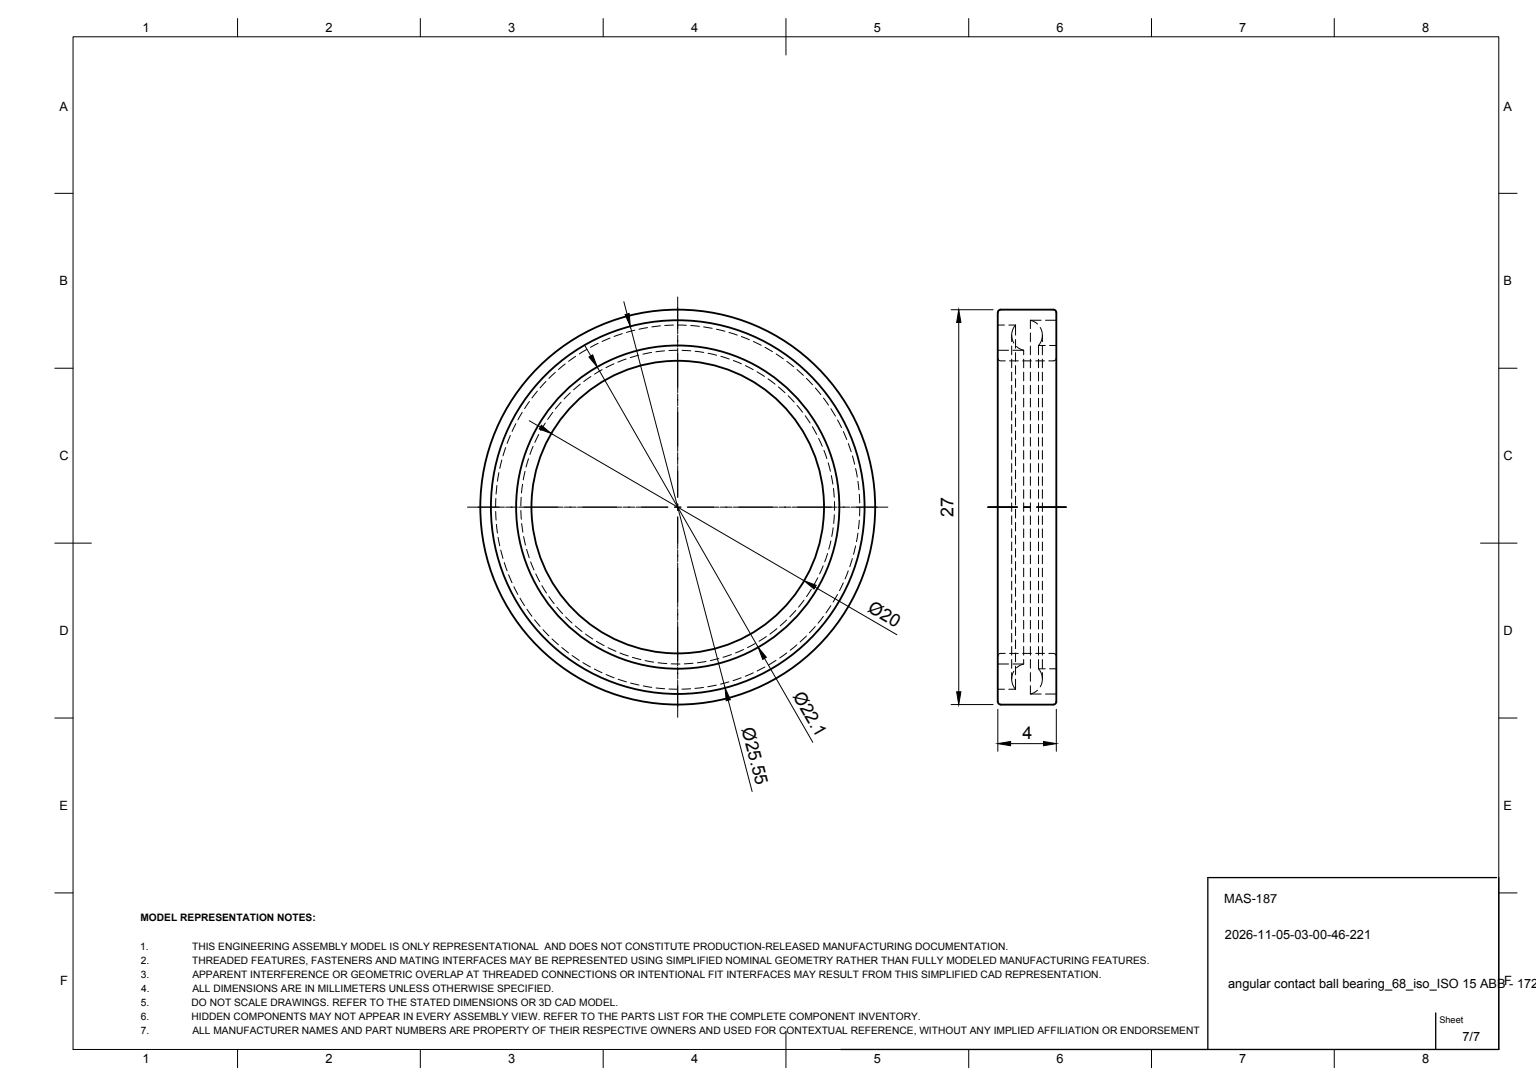
ISO-10303-21;
HEADER;
/* Generated by software containing ST-Developer
 * from STEP Tools, Inc. (www.steptools.com) 
 */

FILE_DESCRIPTION(
/* description */ ('STEP AP214'),
/* implementation_level */ '2;1');

FILE_NAME(
/* name */ 'angular contact ball bearing_68_iso_ISO 15 ABB - 1720 - 28,SI,NC,28_6_8.step',
/* time_stamp */ '2026-11-04T19:00:26-08:00',
/* author */ (''),
/* organization */ (''),
/* preprocessor_version */ 'ST-DEVELOPER v20.2',
/* originating_system */ 'Autodesk Translation Framework v15.17.0.0',
/* authorisation */ '');

FILE_SCHEMA (('AUTOMOTIVE_DESIGN { 1 0 10303 214 3 1 1 }'));
ENDSEC;

DATA;
#10=MECHANICAL_DESIGN_GEOMETRIC_PRESENTATION_REPRESENTATION('',(#274),#5689);
#248=TOROIDAL_SURFACE('',#3187,13.3,0.200000000000003);
#249=TOROIDAL_SURFACE('',#3193,13.3,0.200000000000003);
#250=TOROIDAL_SURFACE('',#3204,11.75,1.05);
#251=TOROIDAL_SURFACE('',#3208,10.2,0.200000000000003);
#252=TOROIDAL_SURFACE('',#3214,10.2,0.200000000000003);
#253=TOROIDAL_SURFACE('',#3223,11.75,1.05);
#260=SHAPE_REPRESENTATION_RELATIONSHIP('SRR','None',#5761,#267);
#267=ADVANCED_BREP_SHAPE_REPRESENTATION('',(#281),#5685);
#274=STYLED_ITEM('',(#5805),#281);
#281=MANIFOLD_SOLID_BREP('Body1',#2964);
#331=FACE_BOUND('',#748,.T.);
#332=FACE_BOUND('',#750,.T.);
#333=FACE_BOUND('',#752,.T.);
#334=FACE_BOUND('',#754,.T.);
#411=PLANE('',#3225);
#412=PLANE('',#3226);
#413=PLANE('',#3227);
#414=PLANE('',#3228);
#530=FACE_OUTER_BOUND('',#735,.T.);
#531=FACE_OUTER_BOUND('',#736,.T.);
#532=FACE_OUTER_BOUND('',#737,.T.);
#533=FACE_OUTER_BOUND('',#738,.T.);
#534=FACE_OUTER_BOUND('',#739,.T.);
#535=FACE_OUTER_BOUND('',#740,.T.);
#536=FACE_OUTER_BOUND('',#741,.T.);
#537=FACE_OUTER_BOUND('',#742,.T.);
#538=FACE_OUTER_BOUND('',#743,.T.);
#539=FACE_OUTER_BOUND('',#744,.T.);
#540=FACE_OUTER_BOUND('',#745,.T.);
#541=FACE_OUTER_BOUND('',#746,.T.);
#542=FACE_OUTER_BOUND('',#747,.T.);
#543=FACE_OUTER_BOUND('',#749,.T.);
#544=FACE_OUTER_BOUND('',#751,.T.);
#545=FACE_OUTER_BOUND('',#753,.T.);
#735=EDGE_LOOP('',(#2472,#2473,#2474,#2475));
#736=EDGE_LOOP('',(#2476,#2477,#2478,#2479));
#737=EDGE_LOOP('',(#2480,#2481,#2482,#2483));
#738=EDGE_LOOP('',(#2484,#2485,#2486,#2487,#2488));
#739=EDGE_LOOP('',(#2489,#2490,#2491,#2492,#2493));
#740=EDGE_LOOP('',(#2494,#2495,#2496,#2497,#2498,#2499));
#741=EDGE_LOOP('',(#2500,#2501,#2502,#2503));
#742=EDGE_LOOP('',(#2504,#2505,#2506,#2507));
#743=EDGE_LOOP('',(#2508,#2509,#2510,#2511));
#744=EDGE_LOOP('',(#2512,#2513,#2514,#2515,#2516));
#745=EDGE_LOOP('',(#2517,#2518,#2519,#2520,#2521));
#746=EDGE_LOOP('',(#2522,#2523,#2524,#2525,#2526,#2527));
#747=EDGE_LOOP('',(#2528));
#748=EDGE_LOOP('',(#2529));
#749=EDGE_LOOP('',(#2530));
#750=EDGE_LOOP('',(#2531));
#751=EDGE_LOOP('',(#2532));
#752=EDGE_LOOP('',(#2533));
#753=EDGE_LOOP('',(#2534));
#754=EDGE_LOOP('',(#2535));
#1000=LINE('',#4725,#1231);
#1001=LINE('',#4735,#1232);
#1002=LINE('',#4745,#1233);
#1003=LINE('',#4761,#1234);
#1004=LINE('',#4769,#1235);
#1005=LINE('',#4775,#1236);
#1231=VECTOR('',#3843,13.5);
#1232=VECTOR('',#3856,12.775);
#1233=VECTOR('',#3867,12.45);
#1234=VECTOR('',#3888,10.);
#1235=VECTOR('',#3899,11.05);
#1236=VECTOR('',#3906,10.725);
#1328=CIRCLE('',#3188,13.3);
#1329=CIRCLE('',#3189,0.200000000000003);
#1330=CIRCLE('',#3190,13.5);
#1331=CIRCLE('',#3192,13.5);
#1332=CIRCLE('',#3194,0.200000000000003);
#1333=CIRCLE('',#3195,13.3);
#1334=CIRCLE('',#3197,12.775);
#1335=CIRCLE('',#3198,12.775);
#1336=CIRCLE('',#3199,12.775);
#1337=CIRCLE('',#3201,12.45);
#1338=CIRCLE('',#3202,12.45);
#1339=CIRCLE('',#3203,12.45);
#1340=CIRCLE('',#3205,11.05);
#1341=CIRCLE('',#3206,1.05);
#1342=CIRCLE('',#3207,11.05);
#1343=CIRCLE('',#3209,10.2);
#1344=CIRCLE('',#3210,0.200000000000003);
#1345=CIRCLE('',#3211,10.);
#1346=CIRCLE('',#3213,10.);
#1347=CIRCLE('',#3215,0.200000000000003);
#1348=CIRCLE('',#3216,10.2);
#1349=CIRCLE('',#3218,11.05);
#1350=CIRCLE('',#3220,10.725);
#1351=CIRCLE('',#3221,10.725);
#1352=CIRCLE('',#3222,10.725);
#1353=CIRCLE('',#3224,1.05);
#1543=VERTEX_POINT('',#4718);
#1544=VERTEX_POINT('',#4720);
#1545=VERTEX_POINT('',#4724);
#1546=VERTEX_POINT('',#4728);
#1547=VERTEX_POINT('',#4732);
#1548=VERTEX_POINT('',#4734);
#1549=VERTEX_POINT('',#4736);
#1550=VERTEX_POINT('',#4740);
#1551=VERTEX_POINT('',#4741);
#1552=VERTEX_POINT('',#4744);
#1553=VERTEX_POINT('',#4748);
#1554=VERTEX_POINT('',#4749);
#1555=VERTEX_POINT('',#4754);
#1556=VERTEX_POINT('',#4756);
#1557=VERTEX_POINT('',#4760);
#1558=VERTEX_POINT('',#4764);
#1559=VERTEX_POINT('',#4768);
#1560=VERTEX_POINT('',#4772);
#1561=VERTEX_POINT('',#4774);
#1562=VERTEX_POINT('',#4776);
#1864=EDGE_CURVE('',#1543,#1543,#1328,.T.);
#1865=EDGE_CURVE('',#1543,#1544,#1329,.T.);
#1866=EDGE_CURVE('',#1544,#1544,#1330,.T.);
#1867=EDGE_CURVE('',#1544,#1545,#1000,.T.);
#1868=EDGE_CURVE('',#1545,#1545,#1331,.T.);
#1869=EDGE_CURVE('',#1545,#1546,#1332,.T.);
#1870=EDGE_CURVE('',#1546,#1546,#1333,.T.);
#1871=EDGE_CURVE('',#1547,#1547,#1334,.T.);
#1872=EDGE_CURVE('',#1547,#1548,#1001,.T.);
#1873=EDGE_CURVE('',#1549,#1548,#1335,.T.);
#1874=EDGE_CURVE('',#1548,#1549,#1336,.T.);
#1875=EDGE_CURVE('',#1550,#1551,#1337,.T.);
#1876=EDGE_CURVE('',#1551,#1550,#1338,.T.);
#1877=EDGE_CURVE('',#1551,#1552,#1002,.T.);
#1878=EDGE_CURVE('',#1552,#1552,#1339,.T.);
#1879=EDGE_CURVE('',#1553,#1554,#1340,.T.);
#1880=EDGE_CURVE('',#1554,#1549,#1341,.T.);
#1881=EDGE_CURVE('',#1554,#1553,#1342,.T.);
#1882=EDGE_CURVE('',#1555,#1555,#1343,.T.);
#1883=EDGE_CURVE('',#1555,#1556,#1344,.T.);
#1884=EDGE_CURVE('',#1556,#1556,#1345,.T.);
#1885=EDGE_CURVE('',#1556,#1557,#1003,.T.);
#1886=EDGE_CURVE('',#1557,#1557,#1346,.T.);
#1887=EDGE_CURVE('',#1557,#1558,#1347,.T.);
#1888=EDGE_CURVE('',#1558,#1558,#1348,.T.);
#1889=EDGE_CURVE('',#1553,#1559,#1004,.T.);
#1890=EDGE_CURVE('',#1559,#1559,#1349,.T.);
#1891=EDGE_CURVE('',#1560,#1560,#1350,.T.);
#1892=EDGE_CURVE('',#1560,#1561,#1005,.T.);
#1893=EDGE_CURVE('',#1562,#1561,#1351,.T.);
#1894=EDGE_CURVE('',#1561,#1562,#1352,.T.);
#1895=EDGE_CURVE('',#1550,#1562,#1353,.T.);
#2472=ORIENTED_EDGE('',*,*,#1864,.F.);
#2473=ORIENTED_EDGE('',*,*,#1865,.T.);
#2474=ORIENTED_EDGE('',*,*,#1866,.T.);
#2475=ORIENTED_EDGE('',*,*,#1865,.F.);
#2476=ORIENTED_EDGE('',*,*,#1866,.F.);
#2477=ORIENTED_EDGE('',*,*,#1867,.T.);
#2478=ORIENTED_EDGE('',*,*,#1868,.T.);
#2479=ORIENTED_EDGE('',*,*,#1867,.F.);
#2480=ORIENTED_EDGE('',*,*,#1868,.F.);
#2481=ORIENTED_EDGE('',*,*,#1869,.T.);
#2482=ORIENTED_EDGE('',*,*,#1870,.T.);
#2483=ORIENTED_EDGE('',*,*,#1869,.F.);
#2484=ORIENTED_EDGE('',*,*,#1871,.F.);
#2485=ORIENTED_EDGE('',*,*,#1872,.T.);
#2486=ORIENTED_EDGE('',*,*,#1873,.F.);
#2487=ORIENTED_EDGE('',*,*,#1874,.F.);
#2488=ORIENTED_EDGE('',*,*,#1872,.F.);
#2489=ORIENTED_EDGE('',*,*,#1875,.F.);
#2490=ORIENTED_EDGE('',*,*,#1876,.F.);
#2491=ORIENTED_EDGE('',*,*,#1877,.T.);
#2492=ORIENTED_EDGE('',*,*,#1878,.T.);
#2493=ORIENTED_EDGE('',*,*,#1877,.F.);
#2494=ORIENTED_EDGE('',*,*,#1879,.T.);
#2495=ORIENTED_EDGE('',*,*,#1880,.T.);
#2496=ORIENTED_EDGE('',*,*,#1873,.T.);
#2497=ORIENTED_EDGE('',*,*,#1874,.T.);
#2498=ORIENTED_EDGE('',*,*,#1880,.F.);
#2499=ORIENTED_EDGE('',*,*,#1881,.T.);
#2500=ORIENTED_EDGE('',*,*,#1882,.F.);
#2501=ORIENTED_EDGE('',*,*,#1883,.T.);
#2502=ORIENTED_EDGE('',*,*,#1884,.T.);
#2503=ORIENTED_EDGE('',*,*,#1883,.F.);
#2504=ORIENTED_EDGE('',*,*,#1884,.F.);
#2505=ORIENTED_EDGE('',*,*,#1885,.T.);
#2506=ORIENTED_EDGE('',*,*,#1886,.T.);
#2507=ORIENTED_EDGE('',*,*,#1885,.F.);
#2508=ORIENTED_EDGE('',*,*,#1886,.F.);
#2509=ORIENTED_EDGE('',*,*,#1887,.T.);
#2510=ORIENTED_EDGE('',*,*,#1888,.T.);
#2511=ORIENTED_EDGE('',*,*,#1887,.F.);
#2512=ORIENTED_EDGE('',*,*,#1879,.F.);
#2513=ORIENTED_EDGE('',*,*,#1889,.T.);
#2514=ORIENTED_EDGE('',*,*,#1890,.T.);
#2515=ORIENTED_EDGE('',*,*,#1889,.F.);
#2516=ORIENTED_EDGE('',*,*,#1881,.F.);
#2517=ORIENTED_EDGE('',*,*,#1891,.F.);
#2518=ORIENTED_EDGE('',*,*,#1892,.T.);
#2519=ORIENTED_EDGE('',*,*,#1893,.F.);
#2520=ORIENTED_EDGE('',*,*,#1894,.F.);
#2521=ORIENTED_EDGE('',*,*,#1892,.F.);
#2522=ORIENTED_EDGE('',*,*,#1875,.T.);
#2523=ORIENTED_EDGE('',*,*,#1876,.T.);
#2524=ORIENTED_EDGE('',*,*,#1895,.T.);
#2525=ORIENTED_EDGE('',*,*,#1893,.T.);
#2526=ORIENTED_EDGE('',*,*,#1894,.T.);
#2527=ORIENTED_EDGE('',*,*,#1895,.F.);
#2528=ORIENTED_EDGE('',*,*,#1891,.T.);
#2529=ORIENTED_EDGE('',*,*,#1888,.F.);
#2530=ORIENTED_EDGE('',*,*,#1890,.F.);
#2531=ORIENTED_EDGE('',*,*,#1882,.T.);
#2532=ORIENTED_EDGE('',*,*,#1864,.T.);
#2533=ORIENTED_EDGE('',*,*,#1878,.F.);
#2534=ORIENTED_EDGE('',*,*,#1870,.F.);
#2535=ORIENTED_EDGE('',*,*,#1871,.T.);
#2788=CYLINDRICAL_SURFACE('',#3191,13.5);
#2789=CYLINDRICAL_SURFACE('',#3196,12.775);
#2790=CYLINDRICAL_SURFACE('',#3200,12.45);
#2791=CYLINDRICAL_SURFACE('',#3212,10.);
#2792=CYLINDRICAL_SURFACE('',#3217,11.05);
#2793=CYLINDRICAL_SURFACE('',#3219,10.725);
#2890=ADVANCED_FACE('',(#530),#248,.T.);
#2891=ADVANCED_FACE('',(#531),#2788,.T.);
#2892=ADVANCED_FACE('',(#532),#249,.T.);
#2893=ADVANCED_FACE('',(#533),#2789,.F.);
#2894=ADVANCED_FACE('',(#534),#2790,.F.);
#2895=ADVANCED_FACE('',(#535),#250,.T.);
#2896=ADVANCED_FACE('',(#536),#251,.T.);
#2897=ADVANCED_FACE('',(#537),#2791,.F.);
#2898=ADVANCED_FACE('',(#538),#252,.T.);
#2899=ADVANCED_FACE('',(#539),#2792,.T.);
#2900=ADVANCED_FACE('',(#540),#2793,.T.);
#2901=ADVANCED_FACE('',(#541),#253,.T.);
#2902=ADVANCED_FACE('',(#542,#331),#411,.T.);
#2903=ADVANCED_FACE('',(#543,#332),#412,.T.);
#2904=ADVANCED_FACE('',(#544,#333),#413,.T.);
#2905=ADVANCED_FACE('',(#545,#334),#414,.T.);
#2964=CLOSED_SHELL('',(#2890,#2891,#2892,#2893,#2894,#2895,#2896,#2897,
#2898,#2899,#2900,#2901,#2902,#2903,#2904,#2905));
#3186=AXIS2_PLACEMENT_3D('',#4716,#3831,#3832);
#3187=AXIS2_PLACEMENT_3D('',#4717,#3833,#3834);
#3188=AXIS2_PLACEMENT_3D('',#4719,#3835,#3836);
#3189=AXIS2_PLACEMENT_3D('',#4721,#3837,#3838);
#3190=AXIS2_PLACEMENT_3D('',#4722,#3839,#3840);
#3191=AXIS2_PLACEMENT_3D('',#4723,#3841,#3842);
#3192=AXIS2_PLACEMENT_3D('',#4726,#3844,#3845);
#3193=AXIS2_PLACEMENT_3D('',#4727,#3846,#3847);
#3194=AXIS2_PLACEMENT_3D('',#4729,#3848,#3849);
#3195=AXIS2_PLACEMENT_3D('',#4730,#3850,#3851);
#3196=AXIS2_PLACEMENT_3D('',#4731,#3852,#3853);
#3197=AXIS2_PLACEMENT_3D('',#4733,#3854,#3855);
#3198=AXIS2_PLACEMENT_3D('',#4737,#3857,#3858);
#3199=AXIS2_PLACEMENT_3D('',#4738,#3859,#3860);
#3200=AXIS2_PLACEMENT_3D('',#4739,#3861,#3862);
#3201=AXIS2_PLACEMENT_3D('',#4742,#3863,#3864);
#3202=AXIS2_PLACEMENT_3D('',#4743,#3865,#3866);
#3203=AXIS2_PLACEMENT_3D('',#4746,#3868,#3869);
#3204=AXIS2_PLACEMENT_3D('',#4747,#3870,#3871);
#3205=AXIS2_PLACEMENT_3D('',#4750,#3872,#3873);
#3206=AXIS2_PLACEMENT_3D('',#4751,#3874,#3875);
#3207=AXIS2_PLACEMENT_3D('',#4752,#3876,#3877);
#3208=AXIS2_PLACEMENT_3D('',#4753,#3878,#3879);
#3209=AXIS2_PLACEMENT_3D('',#4755,#3880,#3881);
#3210=AXIS2_PLACEMENT_3D('',#4757,#3882,#3883);
#3211=AXIS2_PLACEMENT_3D('',#4758,#3884,#3885);
#3212=AXIS2_PLACEMENT_3D('',#4759,#3886,#3887);
#3213=AXIS2_PLACEMENT_3D('',#4762,#3889,#3890);
#3214=AXIS2_PLACEMENT_3D('',#4763,#3891,#3892);
#3215=AXIS2_PLACEMENT_3D('',#4765,#3893,#3894);
#3216=AXIS2_PLACEMENT_3D('',#4766,#3895,#3896);
#3217=AXIS2_PLACEMENT_3D('',#4767,#3897,#3898);
#3218=AXIS2_PLACEMENT_3D('',#4770,#3900,#3901);
#3219=AXIS2_PLACEMENT_3D('',#4771,#3902,#3903);
#3220=AXIS2_PLACEMENT_3D('',#4773,#3904,#3905);
#3221=AXIS2_PLACEMENT_3D('',#4777,#3907,#3908);
#3222=AXIS2_PLACEMENT_3D('',#4778,#3909,#3910);
#3223=AXIS2_PLACEMENT_3D('',#4779,#3911,#3912);
#3224=AXIS2_PLACEMENT_3D('',#4780,#3913,#3914);
#3225=AXIS2_PLACEMENT_3D('',#4781,#3915,#3916);
#3226=AXIS2_PLACEMENT_3D('',#4782,#3917,#3918);
#3227=AXIS2_PLACEMENT_3D('',#4783,#3919,#3920);
#3228=AXIS2_PLACEMENT_3D('',#4784,#3921,#3922);
#3831=DIRECTION('axis',(0.,0.,1.));
#3832=DIRECTION('refdir',(1.,0.,0.));
#3833=DIRECTION('center_axis',(1.,0.,0.));
#3834=DIRECTION('ref_axis',(0.,0.,-1.));
#3835=DIRECTION('center_axis',(1.,0.,0.));
#3836=DIRECTION('ref_axis',(0.,0.,-1.));
#3837=DIRECTION('center_axis',(0.,-1.,-1.22464679914735E-16));
#3838=DIRECTION('ref_axis',(0.,-1.22464679914735E-16,1.));
#3839=DIRECTION('center_axis',(1.,0.,0.));
#3840=DIRECTION('ref_axis',(0.,0.,-1.));
#3841=DIRECTION('center_axis',(1.,0.,0.));
#3842=DIRECTION('ref_axis',(0.,0.,-1.));
#3843=DIRECTION('',(-1.,0.,0.));
#3844=DIRECTION('center_axis',(1.,0.,0.));
#3845=DIRECTION('ref_axis',(0.,0.,-1.));
#3846=DIRECTION('center_axis',(1.,0.,0.));
#3847=DIRECTION('ref_axis',(0.,0.,-1.));
#3848=DIRECTION('center_axis',(0.,-1.,-1.22464679914735E-16));
#3849=DIRECTION('ref_axis',(0.,-1.22464679914735E-16,1.));
#3850=DIRECTION('center_axis',(1.,0.,0.));
#3851=DIRECTION('ref_axis',(0.,0.,-1.));
#3852=DIRECTION('center_axis',(1.,0.,0.));
#3853=DIRECTION('ref_axis',(0.,0.,-1.));
#3854=DIRECTION('center_axis',(1.,0.,0.));
#3855=DIRECTION('ref_axis',(0.,0.,-1.));
#3856=DIRECTION('',(1.,0.,0.));
#3857=DIRECTION('center_axis',(-1.,0.,0.));
#3858=DIRECTION('ref_axis',(0.,0.,-1.));
#3859=DIRECTION('center_axis',(-1.,0.,0.));
#3860=DIRECTION('ref_axis',(0.,0.,-1.));
#3861=DIRECTION('center_axis',(1.,0.,0.));
#3862=DIRECTION('ref_axis',(0.,0.,-1.));
#3863=DIRECTION('center_axis',(1.,0.,0.));
#3864=DIRECTION('ref_axis',(0.,0.,1.));
#3865=DIRECTION('center_axis',(1.,0.,0.));
#3866=DIRECTION('ref_axis',(0.,0.,1.));
#3867=DIRECTION('',(1.,0.,0.));
#3868=DIRECTION('center_axis',(1.,0.,0.));
#3869=DIRECTION('ref_axis',(0.,0.,-1.));
#3870=DIRECTION('center_axis',(-1.,0.,0.));
#3871=DIRECTION('ref_axis',(0.,0.,1.));
#3872=DIRECTION('center_axis',(1.,0.,0.));
#3873=DIRECTION('ref_axis',(0.,0.,-1.));
#3874=DIRECTION('center_axis',(0.,-1.,1.22464679914735E-16));
#3875=DIRECTION('ref_axis',(0.,-1.22464679914735E-16,-1.));
#3876=DIRECTION('center_axis',(1.,0.,0.));
#3877=DIRECTION('ref_axis',(0.,0.,-1.));
#3878=DIRECTION('center_axis',(1.,0.,0.));
#3879=DIRECTION('ref_axis',(0.,0.,-1.));
#3880=DIRECTION('center_axis',(1.,0.,0.));
#3881=DIRECTION('ref_axis',(0.,0.,-1.));
#3882=DIRECTION('center_axis',(0.,-1.,-1.22464679914735E-16));
#3883=DIRECTION('ref_axis',(0.,-1.22464679914735E-16,1.));
#3884=DIRECTION('center_axis',(1.,0.,0.));
#3885=DIRECTION('ref_axis',(0.,0.,-1.));
#3886=DIRECTION('center_axis',(1.,0.,0.));
#3887=DIRECTION('ref_axis',(0.,0.,-1.));
#3888=DIRECTION('',(1.,0.,0.));
#3889=DIRECTION('center_axis',(1.,0.,0.));
#3890=DIRECTION('ref_axis',(0.,0.,-1.));
#3891=DIRECTION('center_axis',(1.,0.,0.));
#3892=DIRECTION('ref_axis',(0.,0.,-1.));
#3893=DIRECTION('center_axis',(0.,-1.,-1.22464679914735E-16));
#3894=DIRECTION('ref_axis',(0.,-1.22464679914735E-16,1.));
#3895=DIRECTION('center_axis',(1.,0.,0.));
#3896=DIRECTION('ref_axis',(0.,0.,-1.));
#3897=DIRECTION('center_axis',(1.,0.,0.));
#3898=DIRECTION('ref_axis',(0.,0.,-1.));
#3899=DIRECTION('',(-1.,0.,0.));
#3900=DIRECTION('center_axis',(1.,0.,0.));
#3901=DIRECTION('ref_axis',(0.,0.,-1.));
#3902=DIRECTION('center_axis',(1.,0.,0.));
#3903=DIRECTION('ref_axis',(0.,0.,-1.));
#3904=DIRECTION('center_axis',(1.,0.,0.));
#3905=DIRECTION('ref_axis',(0.,0.,-1.));
#3906=DIRECTION('',(-1.,0.,0.));
#3907=DIRECTION('center_axis',(-1.,0.,0.));
#3908=DIRECTION('ref_axis',(0.,0.,1.));
#3909=DIRECTION('center_axis',(-1.,0.,0.));
#3910=DIRECTION('ref_axis',(0.,0.,1.));
#3911=DIRECTION('center_axis',(-1.,0.,0.));
#3912=DIRECTION('ref_axis',(0.,0.,1.));
#3913=DIRECTION('center_axis',(0.,-1.,1.22464679914735E-16));
#3914=DIRECTION('ref_axis',(0.,-1.22464679914735E-16,-1.));
#3915=DIRECTION('center_axis',(1.,0.,0.));
#3916=DIRECTION('ref_axis',(0.,0.,-1.));
#3917=DIRECTION('center_axis',(-1.,0.,0.));
#3918=DIRECTION('ref_axis',(0.,0.,1.));
#3919=DIRECTION('center_axis',(1.,0.,0.));
#3920=DIRECTION('ref_axis',(0.,0.,-1.));
#3921=DIRECTION('center_axis',(-1.,0.,0.));
#3922=DIRECTION('ref_axis',(0.,0.,1.));
#4716=CARTESIAN_POINT('',(0.,0.,0.));
#4717=CARTESIAN_POINT('Origin',(1.8,0.,0.));
#4718=CARTESIAN_POINT('',(2.,-1.62878024286598E-15,13.3));
#4719=CARTESIAN_POINT('Origin',(2.,0.,0.));
#4720=CARTESIAN_POINT('',(1.8,-1.65327317884893E-15,13.5));
#4721=CARTESIAN_POINT('Origin',(1.8,-1.62878024286598E-15,13.3));
#4722=CARTESIAN_POINT('Origin',(1.8,0.,0.));
#4723=CARTESIAN_POINT('Origin',(-20.6375,0.,0.));
#4724=CARTESIAN_POINT('',(-1.80000000000001,-1.65327317884893E-15,13.5));
#4725=CARTESIAN_POINT('',(-20.6375,-1.65327317884893E-15,13.5));
#4726=CARTESIAN_POINT('Origin',(-1.8,0.,0.));
#4727=CARTESIAN_POINT('Origin',(-1.8,0.,0.));
#4728=CARTESIAN_POINT('',(-2.,-1.62878024286598E-15,13.3));
#4729=CARTESIAN_POINT('Origin',(-1.8,-1.62878024286598E-15,13.3));
#4730=CARTESIAN_POINT('Origin',(-2.,0.,0.));
#4731=CARTESIAN_POINT('Origin',(-20.6375,0.,0.));
#4732=CARTESIAN_POINT('',(-2.,-1.56448628591074E-15,12.775));
#4733=CARTESIAN_POINT('Origin',(-2.,0.,0.));
#4734=CARTESIAN_POINT('',(-0.227760839478619,-1.56448628591074E-15,12.775));
#4735=CARTESIAN_POINT('',(-20.6375,-1.56448628591074E-15,12.775));
#4736=CARTESIAN_POINT('',(-0.227760839478618,1.56448628591074E-15,-12.775));
#4737=CARTESIAN_POINT('Origin',(-0.227760839478618,0.,0.));
#4738=CARTESIAN_POINT('Origin',(-0.227760839478618,0.,0.));
#4739=CARTESIAN_POINT('Origin',(-20.6375,0.,0.));
#4740=CARTESIAN_POINT('',(0.782623792124928,1.52468526493845E-15,-12.45));
#4741=CARTESIAN_POINT('',(0.782623792124926,-1.52468526493846E-15,12.45));
#4742=CARTESIAN_POINT('Origin',(0.782623792124928,0.,0.));
#4743=CARTESIAN_POINT('Origin',(0.782623792124928,0.,0.));
#4744=CARTESIAN_POINT('',(2.,-1.52468526493846E-15,12.45));
#4745=CARTESIAN_POINT('',(-20.6375,-1.52468526493846E-15,12.45));
#4746=CARTESIAN_POINT('Origin',(2.,0.,0.));
#4747=CARTESIAN_POINT('Origin',(0.,0.,0.));
#4748=CARTESIAN_POINT('',(-0.782623792124928,1.35323471305783E-15,11.05));
#4749=CARTESIAN_POINT('',(-0.782623792124928,-1.35323471305783E-15,-11.05));
#4750=CARTESIAN_POINT('Origin',(-0.782623792124928,0.,0.));
#4751=CARTESIAN_POINT('Origin',(0.,-1.43895998899814E-15,-11.75));
#4752=CARTESIAN_POINT('Origin',(-0.782623792124928,0.,0.));
#4753=CARTESIAN_POINT('Origin',(-1.8,0.,0.));
#4754=CARTESIAN_POINT('',(-2.,-1.2491397351303E-15,10.2));
#4755=CARTESIAN_POINT('Origin',(-2.,0.,0.));
#4756=CARTESIAN_POINT('',(-1.8,-1.22464679914735E-15,10.));
#4757=CARTESIAN_POINT('Origin',(-1.8,-1.2491397351303E-15,10.2));
#4758=CARTESIAN_POINT('Origin',(-1.8,0.,0.));
#4759=CARTESIAN_POINT('Origin',(-20.6375,0.,0.));
#4760=CARTESIAN_POINT('',(1.8,-1.22464679914735E-15,10.));
#4761=CARTESIAN_POINT('',(-20.6375,-1.22464679914735E-15,10.));
#4762=CARTESIAN_POINT('Origin',(1.8,0.,0.));
#4763=CARTESIAN_POINT('Origin',(1.8,0.,0.));
#4764=CARTESIAN_POINT('',(2.,-1.2491397351303E-15,10.2));
#4765=CARTESIAN_POINT('Origin',(1.8,-1.2491397351303E-15,10.2));
#4766=CARTESIAN_POINT('Origin',(2.,0.,0.));
#4767=CARTESIAN_POINT('Origin',(-20.6375,0.,0.));
#4768=CARTESIAN_POINT('',(-2.,-1.35323471305783E-15,11.05));
#4769=CARTESIAN_POINT('',(-20.6375,-1.35323471305783E-15,11.05));
#4770=CARTESIAN_POINT('Origin',(-2.,0.,0.));
#4771=CARTESIAN_POINT('Origin',(-20.6375,0.,0.));
#4772=CARTESIAN_POINT('',(2.,-1.31343369208554E-15,10.725));
#4773=CARTESIAN_POINT('Origin',(2.,0.,0.));
#4774=CARTESIAN_POINT('',(0.227760839478619,-1.31343369208554E-15,10.725));
#4775=CARTESIAN_POINT('',(-20.6375,-1.31343369208554E-15,10.725));
#4776=CARTESIAN_POINT('',(0.227760839478618,1.419059478512E-15,-10.725));
#4777=CARTESIAN_POINT('Origin',(0.227760839478618,0.,0.));
#4778=CARTESIAN_POINT('Origin',(0.227760839478618,0.,0.));
#4779=CARTESIAN_POINT('Origin',(0.,0.,0.));
#4780=CARTESIAN_POINT('Origin',(0.,-1.43895998899814E-15,-11.75));
#4781=CARTESIAN_POINT('Origin',(2.,10.2,0.));
#4782=CARTESIAN_POINT('Origin',(-2.,11.05,0.));
#4783=CARTESIAN_POINT('Origin',(2.,13.3,0.));
#4784=CARTESIAN_POINT('Origin',(-2.,12.775,0.));
#5676=UNCERTAINTY_MEASURE_WITH_UNIT(LENGTH_MEASURE(0.01),#5690,
'DISTANCE_ACCURACY_VALUE',
'Maximum model space distance between geometric entities at asserted c
onnectivities');
#5680=UNCERTAINTY_MEASURE_WITH_UNIT(LENGTH_MEASURE(0.01),#5690,
'DISTANCE_ACCURACY_VALUE',
'Maximum model space distance between geometric entities at asserted c
onnectivities');
#5685=(
GEOMETRIC_REPRESENTATION_CONTEXT(3)
GLOBAL_UNCERTAINTY_ASSIGNED_CONTEXT((#5676))
GLOBAL_UNIT_ASSIGNED_CONTEXT((#5690,#5692,#5693))
REPRESENTATION_CONTEXT('','3D')
);
#5689=(
GEOMETRIC_REPRESENTATION_CONTEXT(3)
GLOBAL_UNCERTAINTY_ASSIGNED_CONTEXT((#5680))
GLOBAL_UNIT_ASSIGNED_CONTEXT((#5690,#5692,#5693))
REPRESENTATION_CONTEXT('','3D')
);
#5690=(
LENGTH_UNIT()
NAMED_UNIT(*)
SI_UNIT(.MILLI.,.METRE.)
);
#5692=(
NAMED_UNIT(*)
PLANE_ANGLE_UNIT()
SI_UNIT($,.RADIAN.)
);
#5693=(
NAMED_UNIT(*)
SI_UNIT($,.STERADIAN.)
SOLID_ANGLE_UNIT()
);
#5698=SHAPE_DEFINITION_REPRESENTATION(#5706,#5761);
#5706=PRODUCT_DEFINITION_SHAPE('',$,#5770);
#5761=SHAPE_REPRESENTATION('',(#3186),#5685);
#5765=PRODUCT_DEFINITION_CONTEXT('part definition',#5791,'design');
#5770=PRODUCT_DEFINITION(
'angular contact ball bearing_68_iso_ISO 15 ABB - 1720 - 28,SI,NC,28_6
8',
'angular contact ball bearing_68_iso_ISO 15 ABB - 1720 - 28,SI,NC,28_6
8',#5778,#5765);
#5778=PRODUCT_DEFINITION_FORMATION('',$,#5797);
#5791=APPLICATION_CONTEXT(
'Core Data for Automotive Mechanical Design Process');
#5792=PRODUCT_CONTEXT('part definition',#5791,'mechanical');
#5797=PRODUCT(
'angular contact ball bearing_68_iso_ISO 15 ABB - 1720 - 28,SI,NC,28_6
8',
'angular contact ball bearing_68_iso_ISO 15 ABB - 1720 - 28,SI,NC,28_6
8',$,(#5792));
#5805=PRESENTATION_STYLE_ASSIGNMENT((#5811));
#5811=SURFACE_STYLE_USAGE(.BOTH.,#5817);
#5817=SURFACE_SIDE_STYLE('',(#5823));
#5823=SURFACE_STYLE_FILL_AREA(#5829);
#5829=FILL_AREA_STYLE('Opaque(122,133,145)',(#5835));
#5835=FILL_AREA_STYLE_COLOUR('Opaque(122,133,145)',#5841);
#5841=COLOUR_RGB('Opaque(122,133,145)',0.47843137254902,0.52156862745098,
0.568627450980392);
ENDSEC;
END-ISO-10303-21;
